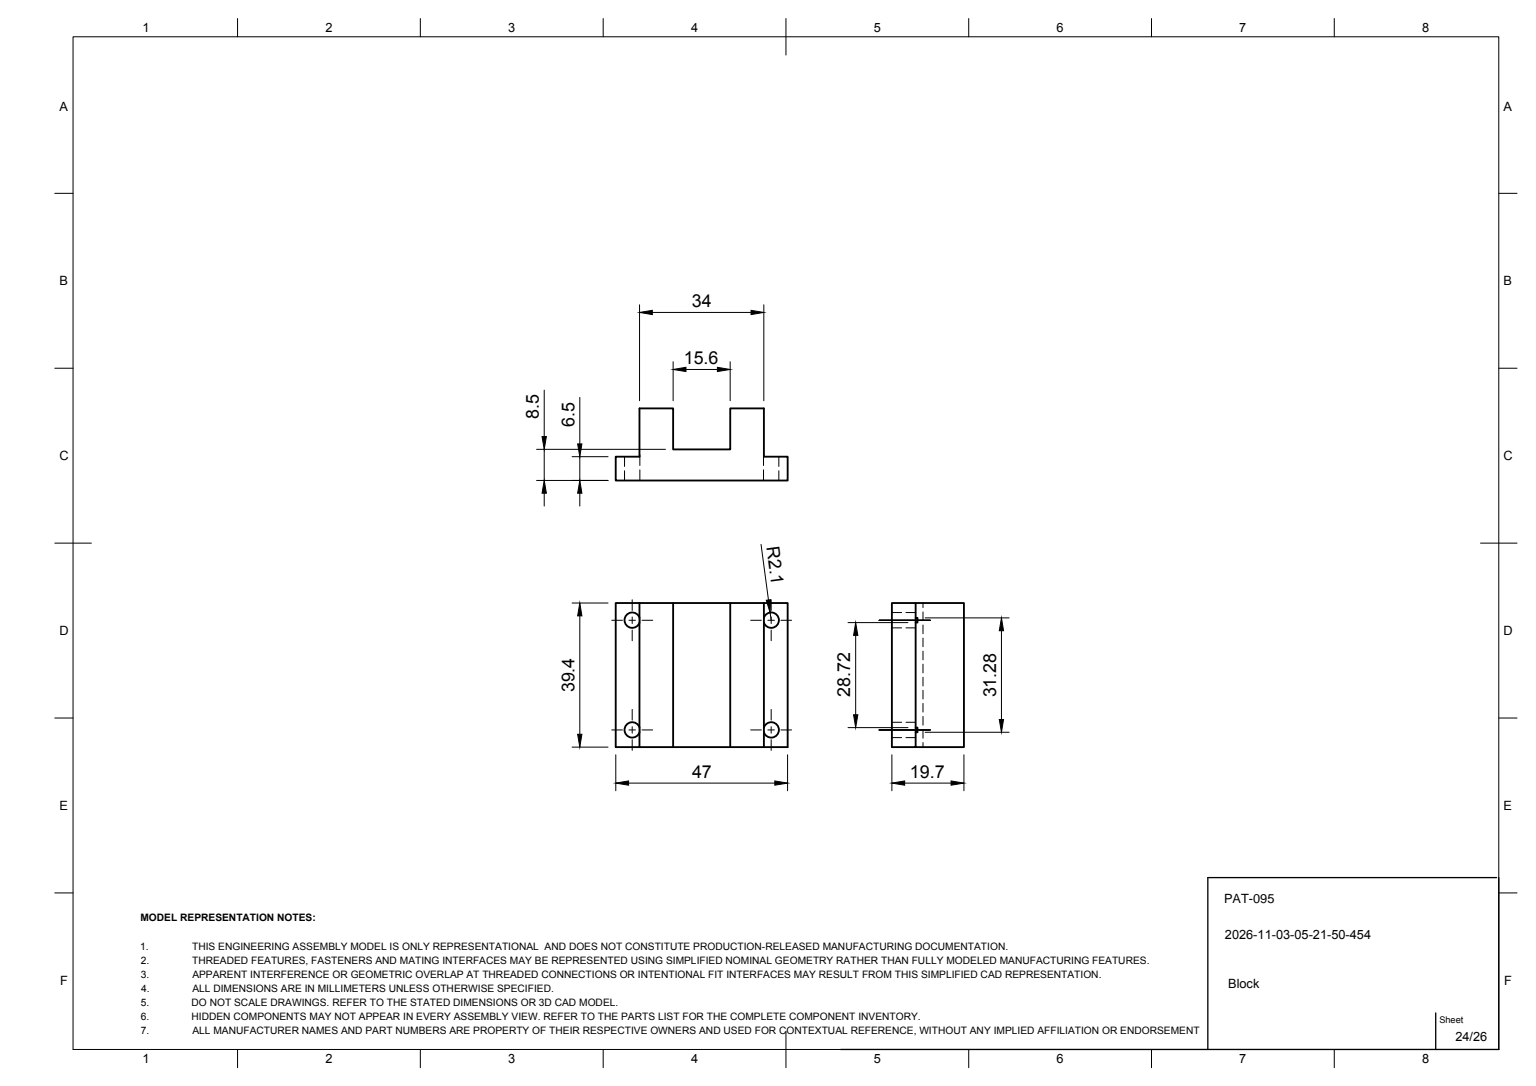
ISO-10303-21;
HEADER;
/* Generated by software containing ST-Developer
 * from STEP Tools, Inc. (www.steptools.com) 
 */

FILE_DESCRIPTION(
/* description */ ('Single-Axis Profile-Rail Linear Slide'),
/* implementation_level */ '2;1');

FILE_NAME(
/* name */ 'Block.step',
/* time_stamp */ '2026-10-27T10:47:43-07:00',
/* author */ (''),
/* organization */ (''),
/* preprocessor_version */ 'ST-DEVELOPER v20.2',
/* originating_system */ 'Autodesk Translation Framework v15.17.0.0',
/* authorisation */ '');

FILE_SCHEMA (('AUTOMOTIVE_DESIGN { 1 0 10303 214 3 1 1 }'));
ENDSEC;

DATA;
#10=MECHANICAL_DESIGN_GEOMETRIC_PRESENTATION_REPRESENTATION('',(#347),#14478);
#293=SHAPE_REPRESENTATION_RELATIONSHIP('SRR','None',#14625,#320);
#320=ADVANCED_BREP_SHAPE_REPRESENTATION('',(#372),#14469);
#347=STYLED_ITEM('',(#14810),#372);
#372=MANIFOLD_SOLID_BREP('Body1',#8609);
#455=FACE_BOUND('',#1734,.T.);
#456=FACE_BOUND('',#1735,.T.);
#457=FACE_BOUND('',#1736,.T.);
#458=FACE_BOUND('',#1737,.T.);
#763=PLANE('',#9394);
#764=PLANE('',#9400);
#765=PLANE('',#9406);
#766=PLANE('',#9412);
#767=PLANE('',#9418);
#768=PLANE('',#9419);
#769=PLANE('',#9420);
#770=PLANE('',#9421);
#771=PLANE('',#9422);
#772=PLANE('',#9423);
#773=PLANE('',#9424);
#774=PLANE('',#9425);
#775=PLANE('',#9426);
#776=PLANE('',#9427);
#777=PLANE('',#9428);
#778=PLANE('',#9429);
#779=PLANE('',#9430);
#780=PLANE('',#9431);
#1188=FACE_OUTER_BOUND('',#1720,.T.);
#1189=FACE_OUTER_BOUND('',#1721,.T.);
#1190=FACE_OUTER_BOUND('',#1722,.T.);
#1191=FACE_OUTER_BOUND('',#1723,.T.);
#1192=FACE_OUTER_BOUND('',#1724,.T.);
#1193=FACE_OUTER_BOUND('',#1725,.T.);
#1194=FACE_OUTER_BOUND('',#1726,.T.);
#1195=FACE_OUTER_BOUND('',#1727,.T.);
#1196=FACE_OUTER_BOUND('',#1728,.T.);
#1197=FACE_OUTER_BOUND('',#1729,.T.);
#1198=FACE_OUTER_BOUND('',#1730,.T.);
#1199=FACE_OUTER_BOUND('',#1731,.T.);
#1200=FACE_OUTER_BOUND('',#1732,.T.);
#1201=FACE_OUTER_BOUND('',#1733,.T.);
#1202=FACE_OUTER_BOUND('',#1738,.T.);
#1203=FACE_OUTER_BOUND('',#1739,.T.);
#1204=FACE_OUTER_BOUND('',#1740,.T.);
#1205=FACE_OUTER_BOUND('',#1741,.T.);
#1206=FACE_OUTER_BOUND('',#1742,.T.);
#1207=FACE_OUTER_BOUND('',#1743,.T.);
#1208=FACE_OUTER_BOUND('',#1744,.T.);
#1209=FACE_OUTER_BOUND('',#1745,.T.);
#1720=EDGE_LOOP('',(#7595,#7596));
#1721=EDGE_LOOP('',(#7597,#7598,#7599,#7600,#7601,#7602,#7603,#7604));
#1722=EDGE_LOOP('',(#7605,#7606));
#1723=EDGE_LOOP('',(#7607,#7608,#7609,#7610,#7611,#7612,#7613,#7614));
#1724=EDGE_LOOP('',(#7615,#7616));
#1725=EDGE_LOOP('',(#7617,#7618,#7619,#7620,#7621,#7622,#7623,#7624));
#1726=EDGE_LOOP('',(#7625,#7626));
#1727=EDGE_LOOP('',(#7627,#7628,#7629,#7630,#7631,#7632,#7633,#7634));
#1728=EDGE_LOOP('',(#7635,#7636,#7637,#7638,#7639,#7640,#7641,#7642,#7643,
#7644,#7645,#7646));
#1729=EDGE_LOOP('',(#7647,#7648,#7649,#7650,#7651,#7652,#7653,#7654,#7655,
#7656,#7657,#7658));
#1730=EDGE_LOOP('',(#7659,#7660,#7661,#7662,#7663,#7664,#7665,#7666,#7667,
#7668,#7669,#7670));
#1731=EDGE_LOOP('',(#7671,#7672,#7673,#7674,#7675,#7676,#7677,#7678,#7679,
#7680));
#1732=EDGE_LOOP('',(#7681,#7682,#7683,#7684));
#1733=EDGE_LOOP('',(#7685,#7686,#7687,#7688));
#1734=EDGE_LOOP('',(#7689));
#1735=EDGE_LOOP('',(#7690));
#1736=EDGE_LOOP('',(#7691));
#1737=EDGE_LOOP('',(#7692));
#1738=EDGE_LOOP('',(#7693,#7694,#7695,#7696));
#1739=EDGE_LOOP('',(#7697,#7698,#7699,#7700,#7701,#7702,#7703,#7704,#7705,
#7706));
#1740=EDGE_LOOP('',(#7707,#7708,#7709,#7710));
#1741=EDGE_LOOP('',(#7711,#7712,#7713,#7714));
#1742=EDGE_LOOP('',(#7715,#7716,#7717,#7718));
#1743=EDGE_LOOP('',(#7719,#7720,#7721,#7722));
#1744=EDGE_LOOP('',(#7723,#7724,#7725,#7726));
#1745=EDGE_LOOP('',(#7727,#7728,#7729,#7730,#7731,#7732,#7733,#7734,#7735,
#7736,#7737,#7738));
#2627=LINE('',#13853,#3598);
#2628=LINE('',#13857,#3599);
#2629=LINE('',#13861,#3600);
#2630=LINE('',#13865,#3601);
#2631=LINE('',#13869,#3602);
#2632=LINE('',#13873,#3603);
#2633=LINE('',#13877,#3604);
#2634=LINE('',#13881,#3605);
#2635=LINE('',#13885,#3606);
#2636=LINE('',#13889,#3607);
#2637=LINE('',#13893,#3608);
#2638=LINE('',#13897,#3609);
#2639=LINE('',#13901,#3610);
#2640=LINE('',#13905,#3611);
#2641=LINE('',#13909,#3612);
#2642=LINE('',#13913,#3613);
#2643=LINE('',#13915,#3614);
#2644=LINE('',#13917,#3615);
#2645=LINE('',#13919,#3616);
#2646=LINE('',#13921,#3617);
#2647=LINE('',#13923,#3618);
#2648=LINE('',#13924,#3619);
#2649=LINE('',#13926,#3620);
#2650=LINE('',#13928,#3621);
#2651=LINE('',#13930,#3622);
#2652=LINE('',#13932,#3623);
#2653=LINE('',#13934,#3624);
#2654=LINE('',#13935,#3625);
#2655=LINE('',#13938,#3626);
#2656=LINE('',#13940,#3627);
#2657=LINE('',#13942,#3628);
#2658=LINE('',#13944,#3629);
#2659=LINE('',#13945,#3630);
#2660=LINE('',#13947,#3631);
#2661=LINE('',#13949,#3632);
#2662=LINE('',#13951,#3633);
#2663=LINE('',#13953,#3634);
#2664=LINE('',#13954,#3635);
#2665=LINE('',#13957,#3636);
#2666=LINE('',#13958,#3637);
#2667=LINE('',#13961,#3638);
#2668=LINE('',#13962,#3639);
#2669=LINE('',#13965,#3640);
#2670=LINE('',#13966,#3641);
#2671=LINE('',#13969,#3642);
#2672=LINE('',#13970,#3643);
#2673=LINE('',#13972,#3644);
#2674=LINE('',#13975,#3645);
#2675=LINE('',#13976,#3646);
#2676=LINE('',#13979,#3647);
#2677=LINE('',#13980,#3648);
#2678=LINE('',#13983,#3649);
#2679=LINE('',#13984,#3650);
#2680=LINE('',#13987,#3651);
#2681=LINE('',#13988,#3652);
#2682=LINE('',#13990,#3653);
#3598=VECTOR('',#11360,1.);
#3599=VECTOR('',#11365,1.);
#3600=VECTOR('',#11368,0.21);
#3601=VECTOR('',#11373,1.);
#3602=VECTOR('',#11376,1.);
#3603=VECTOR('',#11381,1.);
#3604=VECTOR('',#11384,0.21);
#3605=VECTOR('',#11389,1.);
#3606=VECTOR('',#11392,1.);
#3607=VECTOR('',#11397,1.);
#3608=VECTOR('',#11400,0.21);
#3609=VECTOR('',#11405,1.);
#3610=VECTOR('',#11408,1.);
#3611=VECTOR('',#11413,1.);
#3612=VECTOR('',#11416,0.21);
#3613=VECTOR('',#11421,1.);
#3614=VECTOR('',#11424,1.);
#3615=VECTOR('',#11425,1.);
#3616=VECTOR('',#11426,1.);
#3617=VECTOR('',#11427,1.);
#3618=VECTOR('',#11428,1.);
#3619=VECTOR('',#11429,1.);
#3620=VECTOR('',#11432,1.);
#3621=VECTOR('',#11433,1.);
#3622=VECTOR('',#11434,1.);
#3623=VECTOR('',#11435,1.);
#3624=VECTOR('',#11436,1.);
#3625=VECTOR('',#11437,1.);
#3626=VECTOR('',#11440,1.);
#3627=VECTOR('',#11441,1.);
#3628=VECTOR('',#11442,1.);
#3629=VECTOR('',#11443,1.);
#3630=VECTOR('',#11444,1.);
#3631=VECTOR('',#11445,1.);
#3632=VECTOR('',#11446,1.);
#3633=VECTOR('',#11447,1.);
#3634=VECTOR('',#11448,1.);
#3635=VECTOR('',#11449,1.);
#3636=VECTOR('',#11452,1.);
#3637=VECTOR('',#11453,1.);
#3638=VECTOR('',#11456,1.);
#3639=VECTOR('',#11457,1.);
#3640=VECTOR('',#11460,1.);
#3641=VECTOR('',#11461,1.);
#3642=VECTOR('',#11464,1.);
#3643=VECTOR('',#11465,1.);
#3644=VECTOR('',#11468,1.);
#3645=VECTOR('',#11471,1.);
#3646=VECTOR('',#11472,1.);
#3647=VECTOR('',#11475,1.);
#3648=VECTOR('',#11476,1.);
#3649=VECTOR('',#11479,1.);
#3650=VECTOR('',#11480,1.);
#3651=VECTOR('',#11483,1.);
#3652=VECTOR('',#11484,1.);
#3653=VECTOR('',#11487,1.);
#3884=CIRCLE('',#9395,0.21);
#3885=CIRCLE('',#9397,0.21);
#3886=CIRCLE('',#9398,0.21);
#3887=CIRCLE('',#9399,0.21);
#3888=CIRCLE('',#9401,0.21);
#3889=CIRCLE('',#9403,0.21);
#3890=CIRCLE('',#9404,0.21);
#3891=CIRCLE('',#9405,0.21);
#3892=CIRCLE('',#9407,0.21);
#3893=CIRCLE('',#9409,0.21);
#3894=CIRCLE('',#9410,0.21);
#3895=CIRCLE('',#9411,0.21);
#3896=CIRCLE('',#9413,0.21);
#3897=CIRCLE('',#9415,0.21);
#3898=CIRCLE('',#9416,0.21);
#3899=CIRCLE('',#9417,0.21);
#4530=VERTEX_POINT('',#13851);
#4531=VERTEX_POINT('',#13852);
#4532=VERTEX_POINT('',#13856);
#4533=VERTEX_POINT('',#13858);
#4534=VERTEX_POINT('',#13860);
#4535=VERTEX_POINT('',#13863);
#4536=VERTEX_POINT('',#13867);
#4537=VERTEX_POINT('',#13868);
#4538=VERTEX_POINT('',#13872);
#4539=VERTEX_POINT('',#13874);
#4540=VERTEX_POINT('',#13876);
#4541=VERTEX_POINT('',#13879);
#4542=VERTEX_POINT('',#13883);
#4543=VERTEX_POINT('',#13884);
#4544=VERTEX_POINT('',#13888);
#4545=VERTEX_POINT('',#13890);
#4546=VERTEX_POINT('',#13892);
#4547=VERTEX_POINT('',#13895);
#4548=VERTEX_POINT('',#13899);
#4549=VERTEX_POINT('',#13900);
#4550=VERTEX_POINT('',#13904);
#4551=VERTEX_POINT('',#13906);
#4552=VERTEX_POINT('',#13908);
#4553=VERTEX_POINT('',#13911);
#4554=VERTEX_POINT('',#13916);
#4555=VERTEX_POINT('',#13918);
#4556=VERTEX_POINT('',#13920);
#4557=VERTEX_POINT('',#13922);
#4558=VERTEX_POINT('',#13927);
#4559=VERTEX_POINT('',#13929);
#4560=VERTEX_POINT('',#13931);
#4561=VERTEX_POINT('',#13933);
#4562=VERTEX_POINT('',#13937);
#4563=VERTEX_POINT('',#13939);
#4564=VERTEX_POINT('',#13941);
#4565=VERTEX_POINT('',#13943);
#4566=VERTEX_POINT('',#13946);
#4567=VERTEX_POINT('',#13948);
#4568=VERTEX_POINT('',#13950);
#4569=VERTEX_POINT('',#13952);
#4570=VERTEX_POINT('',#13956);
#4571=VERTEX_POINT('',#13960);
#4572=VERTEX_POINT('',#13964);
#4573=VERTEX_POINT('',#13968);
#4574=VERTEX_POINT('',#13974);
#4575=VERTEX_POINT('',#13978);
#4576=VERTEX_POINT('',#13982);
#4577=VERTEX_POINT('',#13986);
#5575=EDGE_CURVE('',#4530,#4531,#2627,.T.);
#5576=EDGE_CURVE('',#4530,#4531,#3884,.T.);
#5577=EDGE_CURVE('',#4532,#4530,#2628,.T.);
#5578=EDGE_CURVE('',#4533,#4532,#3885,.T.);
#5579=EDGE_CURVE('',#4533,#4534,#2629,.T.);
#5580=EDGE_CURVE('',#4534,#4534,#3886,.T.);
#5581=EDGE_CURVE('',#4535,#4533,#3887,.T.);
#5582=EDGE_CURVE('',#4531,#4535,#2630,.T.);
#5583=EDGE_CURVE('',#4536,#4537,#2631,.T.);
#5584=EDGE_CURVE('',#4536,#4537,#3888,.T.);
#5585=EDGE_CURVE('',#4538,#4536,#2632,.T.);
#5586=EDGE_CURVE('',#4539,#4538,#3889,.T.);
#5587=EDGE_CURVE('',#4539,#4540,#2633,.T.);
#5588=EDGE_CURVE('',#4540,#4540,#3890,.T.);
#5589=EDGE_CURVE('',#4541,#4539,#3891,.T.);
#5590=EDGE_CURVE('',#4537,#4541,#2634,.T.);
#5591=EDGE_CURVE('',#4542,#4543,#2635,.T.);
#5592=EDGE_CURVE('',#4542,#4543,#3892,.T.);
#5593=EDGE_CURVE('',#4544,#4542,#2636,.T.);
#5594=EDGE_CURVE('',#4545,#4544,#3893,.T.);
#5595=EDGE_CURVE('',#4545,#4546,#2637,.T.);
#5596=EDGE_CURVE('',#4546,#4546,#3894,.T.);
#5597=EDGE_CURVE('',#4547,#4545,#3895,.T.);
#5598=EDGE_CURVE('',#4543,#4547,#2638,.T.);
#5599=EDGE_CURVE('',#4548,#4549,#2639,.T.);
#5600=EDGE_CURVE('',#4548,#4549,#3896,.T.);
#5601=EDGE_CURVE('',#4550,#4548,#2640,.T.);
#5602=EDGE_CURVE('',#4551,#4550,#3897,.T.);
#5603=EDGE_CURVE('',#4551,#4552,#2641,.T.);
#5604=EDGE_CURVE('',#4552,#4552,#3898,.T.);
#5605=EDGE_CURVE('',#4553,#4551,#3899,.T.);
#5606=EDGE_CURVE('',#4549,#4553,#2642,.T.);
#5607=EDGE_CURVE('',#4535,#4544,#2643,.T.);
#5608=EDGE_CURVE('',#4547,#4554,#2644,.T.);
#5609=EDGE_CURVE('',#4555,#4554,#2645,.T.);
#5610=EDGE_CURVE('',#4555,#4556,#2646,.T.);
#5611=EDGE_CURVE('',#4557,#4556,#2647,.T.);
#5612=EDGE_CURVE('',#4557,#4532,#2648,.T.);
#5613=EDGE_CURVE('',#4541,#4550,#2649,.T.);
#5614=EDGE_CURVE('',#4553,#4558,#2650,.T.);
#5615=EDGE_CURVE('',#4559,#4558,#2651,.T.);
#5616=EDGE_CURVE('',#4560,#4559,#2652,.T.);
#5617=EDGE_CURVE('',#4561,#4560,#2653,.T.);
#5618=EDGE_CURVE('',#4561,#4538,#2654,.T.);
#5619=EDGE_CURVE('',#4554,#4562,#2655,.T.);
#5620=EDGE_CURVE('',#4562,#4563,#2656,.T.);
#5621=EDGE_CURVE('',#4563,#4564,#2657,.T.);
#5622=EDGE_CURVE('',#4564,#4565,#2658,.T.);
#5623=EDGE_CURVE('',#4565,#4561,#2659,.T.);
#5624=EDGE_CURVE('',#4560,#4566,#2660,.T.);
#5625=EDGE_CURVE('',#4566,#4567,#2661,.T.);
#5626=EDGE_CURVE('',#4567,#4568,#2662,.T.);
#5627=EDGE_CURVE('',#4568,#4569,#2663,.T.);
#5628=EDGE_CURVE('',#4569,#4555,#2664,.T.);
#5629=EDGE_CURVE('',#4570,#4557,#2665,.T.);
#5630=EDGE_CURVE('',#4562,#4570,#2666,.T.);
#5631=EDGE_CURVE('',#4571,#4570,#2667,.T.);
#5632=EDGE_CURVE('',#4563,#4571,#2668,.T.);
#5633=EDGE_CURVE('',#4572,#4571,#2669,.T.);
#5634=EDGE_CURVE('',#4564,#4572,#2670,.T.);
#5635=EDGE_CURVE('',#4573,#4572,#2671,.T.);
#5636=EDGE_CURVE('',#4565,#4573,#2672,.T.);
#5637=EDGE_CURVE('',#4558,#4573,#2673,.T.);
#5638=EDGE_CURVE('',#4574,#4559,#2674,.T.);
#5639=EDGE_CURVE('',#4566,#4574,#2675,.T.);
#5640=EDGE_CURVE('',#4575,#4574,#2676,.T.);
#5641=EDGE_CURVE('',#4567,#4575,#2677,.T.);
#5642=EDGE_CURVE('',#4576,#4575,#2678,.T.);
#5643=EDGE_CURVE('',#4568,#4576,#2679,.T.);
#5644=EDGE_CURVE('',#4577,#4576,#2680,.T.);
#5645=EDGE_CURVE('',#4569,#4577,#2681,.T.);
#5646=EDGE_CURVE('',#4556,#4577,#2682,.T.);
#7595=ORIENTED_EDGE('',*,*,#5575,.F.);
#7596=ORIENTED_EDGE('',*,*,#5576,.T.);
#7597=ORIENTED_EDGE('',*,*,#5577,.F.);
#7598=ORIENTED_EDGE('',*,*,#5578,.F.);
#7599=ORIENTED_EDGE('',*,*,#5579,.T.);
#7600=ORIENTED_EDGE('',*,*,#5580,.F.);
#7601=ORIENTED_EDGE('',*,*,#5579,.F.);
#7602=ORIENTED_EDGE('',*,*,#5581,.F.);
#7603=ORIENTED_EDGE('',*,*,#5582,.F.);
#7604=ORIENTED_EDGE('',*,*,#5576,.F.);
#7605=ORIENTED_EDGE('',*,*,#5583,.F.);
#7606=ORIENTED_EDGE('',*,*,#5584,.T.);
#7607=ORIENTED_EDGE('',*,*,#5585,.F.);
#7608=ORIENTED_EDGE('',*,*,#5586,.F.);
#7609=ORIENTED_EDGE('',*,*,#5587,.T.);
#7610=ORIENTED_EDGE('',*,*,#5588,.F.);
#7611=ORIENTED_EDGE('',*,*,#5587,.F.);
#7612=ORIENTED_EDGE('',*,*,#5589,.F.);
#7613=ORIENTED_EDGE('',*,*,#5590,.F.);
#7614=ORIENTED_EDGE('',*,*,#5584,.F.);
#7615=ORIENTED_EDGE('',*,*,#5591,.F.);
#7616=ORIENTED_EDGE('',*,*,#5592,.T.);
#7617=ORIENTED_EDGE('',*,*,#5593,.F.);
#7618=ORIENTED_EDGE('',*,*,#5594,.F.);
#7619=ORIENTED_EDGE('',*,*,#5595,.T.);
#7620=ORIENTED_EDGE('',*,*,#5596,.F.);
#7621=ORIENTED_EDGE('',*,*,#5595,.F.);
#7622=ORIENTED_EDGE('',*,*,#5597,.F.);
#7623=ORIENTED_EDGE('',*,*,#5598,.F.);
#7624=ORIENTED_EDGE('',*,*,#5592,.F.);
#7625=ORIENTED_EDGE('',*,*,#5599,.F.);
#7626=ORIENTED_EDGE('',*,*,#5600,.T.);
#7627=ORIENTED_EDGE('',*,*,#5601,.F.);
#7628=ORIENTED_EDGE('',*,*,#5602,.F.);
#7629=ORIENTED_EDGE('',*,*,#5603,.T.);
#7630=ORIENTED_EDGE('',*,*,#5604,.F.);
#7631=ORIENTED_EDGE('',*,*,#5603,.F.);
#7632=ORIENTED_EDGE('',*,*,#5605,.F.);
#7633=ORIENTED_EDGE('',*,*,#5606,.F.);
#7634=ORIENTED_EDGE('',*,*,#5600,.F.);
#7635=ORIENTED_EDGE('',*,*,#5577,.T.);
#7636=ORIENTED_EDGE('',*,*,#5575,.T.);
#7637=ORIENTED_EDGE('',*,*,#5582,.T.);
#7638=ORIENTED_EDGE('',*,*,#5607,.T.);
#7639=ORIENTED_EDGE('',*,*,#5593,.T.);
#7640=ORIENTED_EDGE('',*,*,#5591,.T.);
#7641=ORIENTED_EDGE('',*,*,#5598,.T.);
#7642=ORIENTED_EDGE('',*,*,#5608,.T.);
#7643=ORIENTED_EDGE('',*,*,#5609,.F.);
#7644=ORIENTED_EDGE('',*,*,#5610,.T.);
#7645=ORIENTED_EDGE('',*,*,#5611,.F.);
#7646=ORIENTED_EDGE('',*,*,#5612,.T.);
#7647=ORIENTED_EDGE('',*,*,#5585,.T.);
#7648=ORIENTED_EDGE('',*,*,#5583,.T.);
#7649=ORIENTED_EDGE('',*,*,#5590,.T.);
#7650=ORIENTED_EDGE('',*,*,#5613,.T.);
#7651=ORIENTED_EDGE('',*,*,#5601,.T.);
#7652=ORIENTED_EDGE('',*,*,#5599,.T.);
#7653=ORIENTED_EDGE('',*,*,#5606,.T.);
#7654=ORIENTED_EDGE('',*,*,#5614,.T.);
#7655=ORIENTED_EDGE('',*,*,#5615,.F.);
#7656=ORIENTED_EDGE('',*,*,#5616,.F.);
#7657=ORIENTED_EDGE('',*,*,#5617,.F.);
#7658=ORIENTED_EDGE('',*,*,#5618,.T.);
#7659=ORIENTED_EDGE('',*,*,#5609,.T.);
#7660=ORIENTED_EDGE('',*,*,#5619,.T.);
#7661=ORIENTED_EDGE('',*,*,#5620,.T.);
#7662=ORIENTED_EDGE('',*,*,#5621,.T.);
#7663=ORIENTED_EDGE('',*,*,#5622,.T.);
#7664=ORIENTED_EDGE('',*,*,#5623,.T.);
#7665=ORIENTED_EDGE('',*,*,#5617,.T.);
#7666=ORIENTED_EDGE('',*,*,#5624,.T.);
#7667=ORIENTED_EDGE('',*,*,#5625,.T.);
#7668=ORIENTED_EDGE('',*,*,#5626,.T.);
#7669=ORIENTED_EDGE('',*,*,#5627,.T.);
#7670=ORIENTED_EDGE('',*,*,#5628,.T.);
#7671=ORIENTED_EDGE('',*,*,#5581,.T.);
#7672=ORIENTED_EDGE('',*,*,#5578,.T.);
#7673=ORIENTED_EDGE('',*,*,#5612,.F.);
#7674=ORIENTED_EDGE('',*,*,#5629,.F.);
#7675=ORIENTED_EDGE('',*,*,#5630,.F.);
#7676=ORIENTED_EDGE('',*,*,#5619,.F.);
#7677=ORIENTED_EDGE('',*,*,#5608,.F.);
#7678=ORIENTED_EDGE('',*,*,#5597,.T.);
#7679=ORIENTED_EDGE('',*,*,#5594,.T.);
#7680=ORIENTED_EDGE('',*,*,#5607,.F.);
#7681=ORIENTED_EDGE('',*,*,#5630,.T.);
#7682=ORIENTED_EDGE('',*,*,#5631,.F.);
#7683=ORIENTED_EDGE('',*,*,#5632,.F.);
#7684=ORIENTED_EDGE('',*,*,#5620,.F.);
#7685=ORIENTED_EDGE('',*,*,#5632,.T.);
#7686=ORIENTED_EDGE('',*,*,#5633,.F.);
#7687=ORIENTED_EDGE('',*,*,#5634,.F.);
#7688=ORIENTED_EDGE('',*,*,#5621,.F.);
#7689=ORIENTED_EDGE('',*,*,#5580,.T.);
#7690=ORIENTED_EDGE('',*,*,#5588,.T.);
#7691=ORIENTED_EDGE('',*,*,#5596,.T.);
#7692=ORIENTED_EDGE('',*,*,#5604,.T.);
#7693=ORIENTED_EDGE('',*,*,#5634,.T.);
#7694=ORIENTED_EDGE('',*,*,#5635,.F.);
#7695=ORIENTED_EDGE('',*,*,#5636,.F.);
#7696=ORIENTED_EDGE('',*,*,#5622,.F.);
#7697=ORIENTED_EDGE('',*,*,#5589,.T.);
#7698=ORIENTED_EDGE('',*,*,#5586,.T.);
#7699=ORIENTED_EDGE('',*,*,#5618,.F.);
#7700=ORIENTED_EDGE('',*,*,#5623,.F.);
#7701=ORIENTED_EDGE('',*,*,#5636,.T.);
#7702=ORIENTED_EDGE('',*,*,#5637,.F.);
#7703=ORIENTED_EDGE('',*,*,#5614,.F.);
#7704=ORIENTED_EDGE('',*,*,#5605,.T.);
#7705=ORIENTED_EDGE('',*,*,#5602,.T.);
#7706=ORIENTED_EDGE('',*,*,#5613,.F.);
#7707=ORIENTED_EDGE('',*,*,#5616,.T.);
#7708=ORIENTED_EDGE('',*,*,#5638,.F.);
#7709=ORIENTED_EDGE('',*,*,#5639,.F.);
#7710=ORIENTED_EDGE('',*,*,#5624,.F.);
#7711=ORIENTED_EDGE('',*,*,#5639,.T.);
#7712=ORIENTED_EDGE('',*,*,#5640,.F.);
#7713=ORIENTED_EDGE('',*,*,#5641,.F.);
#7714=ORIENTED_EDGE('',*,*,#5625,.F.);
#7715=ORIENTED_EDGE('',*,*,#5641,.T.);
#7716=ORIENTED_EDGE('',*,*,#5642,.F.);
#7717=ORIENTED_EDGE('',*,*,#5643,.F.);
#7718=ORIENTED_EDGE('',*,*,#5626,.F.);
#7719=ORIENTED_EDGE('',*,*,#5643,.T.);
#7720=ORIENTED_EDGE('',*,*,#5644,.F.);
#7721=ORIENTED_EDGE('',*,*,#5645,.F.);
#7722=ORIENTED_EDGE('',*,*,#5627,.F.);
#7723=ORIENTED_EDGE('',*,*,#5645,.T.);
#7724=ORIENTED_EDGE('',*,*,#5646,.F.);
#7725=ORIENTED_EDGE('',*,*,#5610,.F.);
#7726=ORIENTED_EDGE('',*,*,#5628,.F.);
#7727=ORIENTED_EDGE('',*,*,#5611,.T.);
#7728=ORIENTED_EDGE('',*,*,#5646,.T.);
#7729=ORIENTED_EDGE('',*,*,#5644,.T.);
#7730=ORIENTED_EDGE('',*,*,#5642,.T.);
#7731=ORIENTED_EDGE('',*,*,#5640,.T.);
#7732=ORIENTED_EDGE('',*,*,#5638,.T.);
#7733=ORIENTED_EDGE('',*,*,#5615,.T.);
#7734=ORIENTED_EDGE('',*,*,#5637,.T.);
#7735=ORIENTED_EDGE('',*,*,#5635,.T.);
#7736=ORIENTED_EDGE('',*,*,#5633,.T.);
#7737=ORIENTED_EDGE('',*,*,#5631,.T.);
#7738=ORIENTED_EDGE('',*,*,#5629,.T.);
#8118=CYLINDRICAL_SURFACE('',#9396,0.21);
#8119=CYLINDRICAL_SURFACE('',#9402,0.21);
#8120=CYLINDRICAL_SURFACE('',#9408,0.21);
#8121=CYLINDRICAL_SURFACE('',#9414,0.21);
#8482=ADVANCED_FACE('',(#1188),#763,.T.);
#8483=ADVANCED_FACE('',(#1189),#8118,.F.);
#8484=ADVANCED_FACE('',(#1190),#764,.T.);
#8485=ADVANCED_FACE('',(#1191),#8119,.F.);
#8486=ADVANCED_FACE('',(#1192),#765,.T.);
#8487=ADVANCED_FACE('',(#1193),#8120,.F.);
#8488=ADVANCED_FACE('',(#1194),#766,.T.);
#8489=ADVANCED_FACE('',(#1195),#8121,.F.);
#8490=ADVANCED_FACE('',(#1196),#767,.T.);
#8491=ADVANCED_FACE('',(#1197),#768,.T.);
#8492=ADVANCED_FACE('',(#1198),#769,.T.);
#8493=ADVANCED_FACE('',(#1199),#770,.T.);
#8494=ADVANCED_FACE('',(#1200),#771,.T.);
#8495=ADVANCED_FACE('',(#1201,#455,#456,#457,#458),#772,.T.);
#8496=ADVANCED_FACE('',(#1202),#773,.T.);
#8497=ADVANCED_FACE('',(#1203),#774,.T.);
#8498=ADVANCED_FACE('',(#1204),#775,.T.);
#8499=ADVANCED_FACE('',(#1205),#776,.T.);
#8500=ADVANCED_FACE('',(#1206),#777,.T.);
#8501=ADVANCED_FACE('',(#1207),#778,.T.);
#8502=ADVANCED_FACE('',(#1208),#779,.T.);
#8503=ADVANCED_FACE('',(#1209),#780,.T.);
#8609=CLOSED_SHELL('',(#8482,#8483,#8484,#8485,#8486,#8487,#8488,#8489,
#8490,#8491,#8492,#8493,#8494,#8495,#8496,#8497,#8498,#8499,#8500,#8501,
#8502,#8503));
#9393=AXIS2_PLACEMENT_3D('',#13849,#11356,#11357);
#9394=AXIS2_PLACEMENT_3D('',#13850,#11358,#11359);
#9395=AXIS2_PLACEMENT_3D('',#13854,#11361,#11362);
#9396=AXIS2_PLACEMENT_3D('',#13855,#11363,#11364);
#9397=AXIS2_PLACEMENT_3D('',#13859,#11366,#11367);
#9398=AXIS2_PLACEMENT_3D('',#13862,#11369,#11370);
#9399=AXIS2_PLACEMENT_3D('',#13864,#11371,#11372);
#9400=AXIS2_PLACEMENT_3D('',#13866,#11374,#11375);
#9401=AXIS2_PLACEMENT_3D('',#13870,#11377,#11378);
#9402=AXIS2_PLACEMENT_3D('',#13871,#11379,#11380);
#9403=AXIS2_PLACEMENT_3D('',#13875,#11382,#11383);
#9404=AXIS2_PLACEMENT_3D('',#13878,#11385,#11386);
#9405=AXIS2_PLACEMENT_3D('',#13880,#11387,#11388);
#9406=AXIS2_PLACEMENT_3D('',#13882,#11390,#11391);
#9407=AXIS2_PLACEMENT_3D('',#13886,#11393,#11394);
#9408=AXIS2_PLACEMENT_3D('',#13887,#11395,#11396);
#9409=AXIS2_PLACEMENT_3D('',#13891,#11398,#11399);
#9410=AXIS2_PLACEMENT_3D('',#13894,#11401,#11402);
#9411=AXIS2_PLACEMENT_3D('',#13896,#11403,#11404);
#9412=AXIS2_PLACEMENT_3D('',#13898,#11406,#11407);
#9413=AXIS2_PLACEMENT_3D('',#13902,#11409,#11410);
#9414=AXIS2_PLACEMENT_3D('',#13903,#11411,#11412);
#9415=AXIS2_PLACEMENT_3D('',#13907,#11414,#11415);
#9416=AXIS2_PLACEMENT_3D('',#13910,#11417,#11418);
#9417=AXIS2_PLACEMENT_3D('',#13912,#11419,#11420);
#9418=AXIS2_PLACEMENT_3D('',#13914,#11422,#11423);
#9419=AXIS2_PLACEMENT_3D('',#13925,#11430,#11431);
#9420=AXIS2_PLACEMENT_3D('',#13936,#11438,#11439);
#9421=AXIS2_PLACEMENT_3D('',#13955,#11450,#11451);
#9422=AXIS2_PLACEMENT_3D('',#13959,#11454,#11455);
#9423=AXIS2_PLACEMENT_3D('',#13963,#11458,#11459);
#9424=AXIS2_PLACEMENT_3D('',#13967,#11462,#11463);
#9425=AXIS2_PLACEMENT_3D('',#13971,#11466,#11467);
#9426=AXIS2_PLACEMENT_3D('',#13973,#11469,#11470);
#9427=AXIS2_PLACEMENT_3D('',#13977,#11473,#11474);
#9428=AXIS2_PLACEMENT_3D('',#13981,#11477,#11478);
#9429=AXIS2_PLACEMENT_3D('',#13985,#11481,#11482);
#9430=AXIS2_PLACEMENT_3D('',#13989,#11485,#11486);
#9431=AXIS2_PLACEMENT_3D('',#13991,#11488,#11489);
#11356=DIRECTION('axis',(0.,0.,1.));
#11357=DIRECTION('refdir',(1.,0.,0.));
#11358=DIRECTION('center_axis',(0.,0.,1.));
#11359=DIRECTION('ref_axis',(1.,0.,0.));
#11360=DIRECTION('',(-1.,0.,0.));
#11361=DIRECTION('center_axis',(0.,0.,1.));
#11362=DIRECTION('ref_axis',(1.,0.,0.));
#11363=DIRECTION('center_axis',(0.,0.,1.));
#11364=DIRECTION('ref_axis',(1.,0.,0.));
#11365=DIRECTION('',(0.,0.,-1.));
#11366=DIRECTION('center_axis',(0.,0.,1.));
#11367=DIRECTION('ref_axis',(1.,0.,0.));
#11368=DIRECTION('',(0.,0.,1.));
#11369=DIRECTION('center_axis',(0.,0.,-1.));
#11370=DIRECTION('ref_axis',(1.,0.,0.));
#11371=DIRECTION('center_axis',(0.,0.,1.));
#11372=DIRECTION('ref_axis',(1.,0.,0.));
#11373=DIRECTION('',(0.,0.,1.));
#11374=DIRECTION('center_axis',(0.,0.,1.));
#11375=DIRECTION('ref_axis',(1.,0.,0.));
#11376=DIRECTION('',(1.,0.,0.));
#11377=DIRECTION('center_axis',(0.,0.,1.));
#11378=DIRECTION('ref_axis',(1.,0.,0.));
#11379=DIRECTION('center_axis',(0.,0.,1.));
#11380=DIRECTION('ref_axis',(1.,0.,0.));
#11381=DIRECTION('',(0.,0.,-1.));
#11382=DIRECTION('center_axis',(0.,0.,1.));
#11383=DIRECTION('ref_axis',(1.,0.,0.));
#11384=DIRECTION('',(0.,0.,1.));
#11385=DIRECTION('center_axis',(0.,0.,-1.));
#11386=DIRECTION('ref_axis',(1.,0.,0.));
#11387=DIRECTION('center_axis',(0.,0.,1.));
#11388=DIRECTION('ref_axis',(1.,0.,0.));
#11389=DIRECTION('',(0.,0.,1.));
#11390=DIRECTION('center_axis',(0.,0.,1.));
#11391=DIRECTION('ref_axis',(1.,0.,0.));
#11392=DIRECTION('',(-1.,0.,0.));
#11393=DIRECTION('center_axis',(0.,0.,1.));
#11394=DIRECTION('ref_axis',(1.,0.,0.));
#11395=DIRECTION('center_axis',(0.,0.,1.));
#11396=DIRECTION('ref_axis',(1.,0.,0.));
#11397=DIRECTION('',(0.,0.,-1.));
#11398=DIRECTION('center_axis',(0.,0.,1.));
#11399=DIRECTION('ref_axis',(1.,0.,0.));
#11400=DIRECTION('',(0.,0.,1.));
#11401=DIRECTION('center_axis',(0.,0.,-1.));
#11402=DIRECTION('ref_axis',(1.,0.,0.));
#11403=DIRECTION('center_axis',(0.,0.,1.));
#11404=DIRECTION('ref_axis',(1.,0.,0.));
#11405=DIRECTION('',(0.,0.,1.));
#11406=DIRECTION('center_axis',(0.,0.,1.));
#11407=DIRECTION('ref_axis',(1.,0.,0.));
#11408=DIRECTION('',(1.,0.,0.));
#11409=DIRECTION('center_axis',(0.,0.,1.));
#11410=DIRECTION('ref_axis',(1.,0.,0.));
#11411=DIRECTION('center_axis',(0.,0.,1.));
#11412=DIRECTION('ref_axis',(1.,0.,0.));
#11413=DIRECTION('',(0.,0.,-1.));
#11414=DIRECTION('center_axis',(0.,0.,1.));
#11415=DIRECTION('ref_axis',(1.,0.,0.));
#11416=DIRECTION('',(0.,0.,1.));
#11417=DIRECTION('center_axis',(0.,0.,-1.));
#11418=DIRECTION('ref_axis',(1.,0.,0.));
#11419=DIRECTION('center_axis',(0.,0.,1.));
#11420=DIRECTION('ref_axis',(1.,0.,0.));
#11421=DIRECTION('',(0.,0.,1.));
#11422=DIRECTION('center_axis',(0.,-1.,0.));
#11423=DIRECTION('ref_axis',(0.,0.,-1.));
#11424=DIRECTION('',(-1.,0.,0.));
#11425=DIRECTION('',(-1.,0.,0.));
#11426=DIRECTION('',(0.,0.,1.));
#11427=DIRECTION('',(1.,0.,0.));
#11428=DIRECTION('',(0.,0.,-1.));
#11429=DIRECTION('',(-1.,0.,0.));
#11430=DIRECTION('center_axis',(0.,1.,0.));
#11431=DIRECTION('ref_axis',(0.,0.,1.));
#11432=DIRECTION('',(1.,0.,0.));
#11433=DIRECTION('',(1.,0.,0.));
#11434=DIRECTION('',(0.,0.,1.));
#11435=DIRECTION('',(1.,0.,0.));
#11436=DIRECTION('',(0.,0.,-1.));
#11437=DIRECTION('',(1.,0.,0.));
#11438=DIRECTION('center_axis',(-1.,0.,0.));
#11439=DIRECTION('ref_axis',(0.,0.,1.));
#11440=DIRECTION('',(0.,-1.,0.));
#11441=DIRECTION('',(0.,0.,1.));
#11442=DIRECTION('',(0.,1.,0.));
#11443=DIRECTION('',(0.,0.,-1.));
#11444=DIRECTION('',(0.,-1.,0.));
#11445=DIRECTION('',(0.,-1.,0.));
#11446=DIRECTION('',(0.,0.,1.));
#11447=DIRECTION('',(0.,-1.,0.));
#11448=DIRECTION('',(0.,0.,-1.));
#11449=DIRECTION('',(0.,-1.,0.));
#11450=DIRECTION('center_axis',(0.,0.,-1.));
#11451=DIRECTION('ref_axis',(0.,1.,0.));
#11452=DIRECTION('',(0.,1.,0.));
#11453=DIRECTION('',(1.,0.,0.));
#11454=DIRECTION('center_axis',(0.,-1.,0.));
#11455=DIRECTION('ref_axis',(0.,0.,-1.));
#11456=DIRECTION('',(0.,0.,-1.));
#11457=DIRECTION('',(1.,0.,0.));
#11458=DIRECTION('center_axis',(0.,0.,1.));
#11459=DIRECTION('ref_axis',(0.,-1.,0.));
#11460=DIRECTION('',(0.,-1.,0.));
#11461=DIRECTION('',(1.,0.,0.));
#11462=DIRECTION('center_axis',(0.,1.,0.));
#11463=DIRECTION('ref_axis',(0.,0.,1.));
#11464=DIRECTION('',(0.,0.,1.));
#11465=DIRECTION('',(1.,0.,0.));
#11466=DIRECTION('center_axis',(0.,0.,-1.));
#11467=DIRECTION('ref_axis',(0.,1.,0.));
#11468=DIRECTION('',(0.,1.,0.));
#11469=DIRECTION('center_axis',(0.,0.,-1.));
#11470=DIRECTION('ref_axis',(0.,1.,0.));
#11471=DIRECTION('',(0.,1.,0.));
#11472=DIRECTION('',(1.,0.,0.));
#11473=DIRECTION('center_axis',(0.,-1.,0.));
#11474=DIRECTION('ref_axis',(0.,0.,-1.));
#11475=DIRECTION('',(0.,0.,-1.));
#11476=DIRECTION('',(1.,0.,0.));
#11477=DIRECTION('center_axis',(0.,0.,-1.));
#11478=DIRECTION('ref_axis',(0.,1.,0.));
#11479=DIRECTION('',(0.,1.,0.));
#11480=DIRECTION('',(1.,0.,0.));
#11481=DIRECTION('center_axis',(0.,1.,0.));
#11482=DIRECTION('ref_axis',(0.,0.,1.));
#11483=DIRECTION('',(0.,0.,1.));
#11484=DIRECTION('',(1.,0.,0.));
#11485=DIRECTION('center_axis',(0.,0.,-1.));
#11486=DIRECTION('ref_axis',(0.,1.,0.));
#11487=DIRECTION('',(0.,1.,0.));
#11488=DIRECTION('center_axis',(1.,0.,0.));
#11489=DIRECTION('ref_axis',(0.,0.,-1.));
#13849=CARTESIAN_POINT('',(0.,0.,0.));
#13850=CARTESIAN_POINT('Origin',(1.5,-1.9,1.7));
#13851=CARTESIAN_POINT('',(1.56403124237433,-1.7,1.7));
#13852=CARTESIAN_POINT('',(1.43596875762567,-1.7,1.7));
#13853=CARTESIAN_POINT('',(0.75,-1.7,1.7));
#13854=CARTESIAN_POINT('Origin',(1.5,-1.9,1.7));
#13855=CARTESIAN_POINT('Origin',(1.5,-1.9,1.7));
#13856=CARTESIAN_POINT('',(1.56403124237433,-1.7,1.75));
#13857=CARTESIAN_POINT('',(1.56403124237433,-1.7,1.7));
#13858=CARTESIAN_POINT('',(1.29,-1.9,1.75));
#13859=CARTESIAN_POINT('Origin',(1.5,-1.9,1.75));
#13860=CARTESIAN_POINT('',(1.29,-1.9,2.4));
#13861=CARTESIAN_POINT('',(1.29,-1.9,1.7));
#13862=CARTESIAN_POINT('Origin',(1.5,-1.9,2.4));
#13863=CARTESIAN_POINT('',(1.43596875762567,-1.7,1.75));
#13864=CARTESIAN_POINT('Origin',(1.5,-1.9,1.75));
#13865=CARTESIAN_POINT('',(1.43596875762567,-1.7,1.7));
#13866=CARTESIAN_POINT('Origin',(-1.5,1.9,1.7));
#13867=CARTESIAN_POINT('',(-1.56403124237433,1.7,1.7));
#13868=CARTESIAN_POINT('',(-1.43596875762567,1.7,1.7));
#13869=CARTESIAN_POINT('',(-0.75,1.7,1.7));
#13870=CARTESIAN_POINT('Origin',(-1.5,1.9,1.7));
#13871=CARTESIAN_POINT('Origin',(-1.5,1.9,1.7));
#13872=CARTESIAN_POINT('',(-1.56403124237433,1.7,1.75));
#13873=CARTESIAN_POINT('',(-1.56403124237433,1.7,1.7));
#13874=CARTESIAN_POINT('',(-1.71,1.9,1.75));
#13875=CARTESIAN_POINT('Origin',(-1.5,1.9,1.75));
#13876=CARTESIAN_POINT('',(-1.71,1.9,2.4));
#13877=CARTESIAN_POINT('',(-1.71,1.9,1.7));
#13878=CARTESIAN_POINT('Origin',(-1.5,1.9,2.4));
#13879=CARTESIAN_POINT('',(-1.43596875762567,1.7,1.75));
#13880=CARTESIAN_POINT('Origin',(-1.5,1.9,1.75));
#13881=CARTESIAN_POINT('',(-1.43596875762567,1.7,1.7));
#13882=CARTESIAN_POINT('Origin',(-1.5,-1.9,1.7));
#13883=CARTESIAN_POINT('',(-1.43596875762567,-1.7,1.7));
#13884=CARTESIAN_POINT('',(-1.56403124237433,-1.7,1.7));
#13885=CARTESIAN_POINT('',(-0.75,-1.7,1.7));
#13886=CARTESIAN_POINT('Origin',(-1.5,-1.9,1.7));
#13887=CARTESIAN_POINT('Origin',(-1.5,-1.9,1.7));
#13888=CARTESIAN_POINT('',(-1.43596875762567,-1.7,1.75));
#13889=CARTESIAN_POINT('',(-1.43596875762567,-1.7,1.7));
#13890=CARTESIAN_POINT('',(-1.71,-1.9,1.75));
#13891=CARTESIAN_POINT('Origin',(-1.5,-1.9,1.75));
#13892=CARTESIAN_POINT('',(-1.71,-1.9,2.4));
#13893=CARTESIAN_POINT('',(-1.71,-1.9,1.7));
#13894=CARTESIAN_POINT('Origin',(-1.5,-1.9,2.4));
#13895=CARTESIAN_POINT('',(-1.56403124237433,-1.7,1.75));
#13896=CARTESIAN_POINT('Origin',(-1.5,-1.9,1.75));
#13897=CARTESIAN_POINT('',(-1.56403124237433,-1.7,1.7));
#13898=CARTESIAN_POINT('Origin',(1.5,1.9,1.7));
#13899=CARTESIAN_POINT('',(1.43596875762567,1.7,1.7));
#13900=CARTESIAN_POINT('',(1.56403124237433,1.7,1.7));
#13901=CARTESIAN_POINT('',(0.75,1.7,1.7));
#13902=CARTESIAN_POINT('Origin',(1.5,1.9,1.7));
#13903=CARTESIAN_POINT('Origin',(1.5,1.9,1.7));
#13904=CARTESIAN_POINT('',(1.43596875762567,1.7,1.75));
#13905=CARTESIAN_POINT('',(1.43596875762567,1.7,1.7));
#13906=CARTESIAN_POINT('',(1.29,1.9,1.75));
#13907=CARTESIAN_POINT('Origin',(1.5,1.9,1.75));
#13908=CARTESIAN_POINT('',(1.29,1.9,2.4));
#13909=CARTESIAN_POINT('',(1.29,1.9,1.7));
#13910=CARTESIAN_POINT('Origin',(1.5,1.9,2.4));
#13911=CARTESIAN_POINT('',(1.56403124237433,1.7,1.75));
#13912=CARTESIAN_POINT('Origin',(1.5,1.9,1.75));
#13913=CARTESIAN_POINT('',(1.56403124237433,1.7,1.7));
#13914=CARTESIAN_POINT('Origin',(0.,-1.7,1.75));
#13915=CARTESIAN_POINT('',(0.,-1.7,1.75));
#13916=CARTESIAN_POINT('',(-1.97,-1.7,1.75));
#13917=CARTESIAN_POINT('',(0.,-1.7,1.75));
#13918=CARTESIAN_POINT('',(-1.97,-1.7,0.43));
#13919=CARTESIAN_POINT('',(-1.97,-1.7,1.75));
#13920=CARTESIAN_POINT('',(1.97,-1.7,0.43));
#13921=CARTESIAN_POINT('',(0.,-1.7,0.43));
#13922=CARTESIAN_POINT('',(1.97,-1.7,1.75));
#13923=CARTESIAN_POINT('',(1.97,-1.7,1.75));
#13924=CARTESIAN_POINT('',(0.,-1.7,1.75));
#13925=CARTESIAN_POINT('Origin',(0.,1.7,0.43));
#13926=CARTESIAN_POINT('',(0.,1.7,1.75));
#13927=CARTESIAN_POINT('',(1.97,1.7,1.75));
#13928=CARTESIAN_POINT('',(0.,1.7,1.75));
#13929=CARTESIAN_POINT('',(1.97,1.7,0.43));
#13930=CARTESIAN_POINT('',(1.97,1.7,0.43));
#13931=CARTESIAN_POINT('',(-1.97,1.7,0.43));
#13932=CARTESIAN_POINT('',(0.,1.7,0.43));
#13933=CARTESIAN_POINT('',(-1.97,1.7,1.75));
#13934=CARTESIAN_POINT('',(-1.97,1.7,0.43));
#13935=CARTESIAN_POINT('',(0.,1.7,1.75));
#13936=CARTESIAN_POINT('Origin',(-1.97,0.,1.415));
#13937=CARTESIAN_POINT('',(-1.97,-2.35,1.75));
#13938=CARTESIAN_POINT('',(-1.97,-2.35,1.75));
#13939=CARTESIAN_POINT('',(-1.97,-2.35,2.4));
#13940=CARTESIAN_POINT('',(-1.97,-2.35,2.4));
#13941=CARTESIAN_POINT('',(-1.97,2.35,2.4));
#13942=CARTESIAN_POINT('',(-1.97,2.35,2.4));
#13943=CARTESIAN_POINT('',(-1.97,2.35,1.75));
#13944=CARTESIAN_POINT('',(-1.97,2.35,1.75));
#13945=CARTESIAN_POINT('',(-1.97,1.7,1.75));
#13946=CARTESIAN_POINT('',(-1.97,0.78,0.43));
#13947=CARTESIAN_POINT('',(-1.97,0.78,0.43));
#13948=CARTESIAN_POINT('',(-1.97,0.78,1.55));
#13949=CARTESIAN_POINT('',(-1.97,0.78,1.55));
#13950=CARTESIAN_POINT('',(-1.97,-0.78,1.55));
#13951=CARTESIAN_POINT('',(-1.97,-0.78,1.55));
#13952=CARTESIAN_POINT('',(-1.97,-0.78,0.43));
#13953=CARTESIAN_POINT('',(-1.97,-0.78,0.43));
#13954=CARTESIAN_POINT('',(-1.97,-1.7,0.43));
#13955=CARTESIAN_POINT('Origin',(0.,-2.35,1.75));
#13956=CARTESIAN_POINT('',(1.97,-2.35,1.75));
#13957=CARTESIAN_POINT('',(1.97,-2.35,1.75));
#13958=CARTESIAN_POINT('',(0.,-2.35,1.75));
#13959=CARTESIAN_POINT('Origin',(0.,-2.35,2.4));
#13960=CARTESIAN_POINT('',(1.97,-2.35,2.4));
#13961=CARTESIAN_POINT('',(1.97,-2.35,2.4));
#13962=CARTESIAN_POINT('',(0.,-2.35,2.4));
#13963=CARTESIAN_POINT('Origin',(0.,2.35,2.4));
#13964=CARTESIAN_POINT('',(1.97,2.35,2.4));
#13965=CARTESIAN_POINT('',(1.97,2.35,2.4));
#13966=CARTESIAN_POINT('',(0.,2.35,2.4));
#13967=CARTESIAN_POINT('Origin',(0.,2.35,1.75));
#13968=CARTESIAN_POINT('',(1.97,2.35,1.75));
#13969=CARTESIAN_POINT('',(1.97,2.35,1.75));
#13970=CARTESIAN_POINT('',(0.,2.35,1.75));
#13971=CARTESIAN_POINT('Origin',(0.,1.7,1.75));
#13972=CARTESIAN_POINT('',(1.97,1.7,1.75));
#13973=CARTESIAN_POINT('Origin',(0.,0.78,0.43));
#13974=CARTESIAN_POINT('',(1.97,0.78,0.43));
#13975=CARTESIAN_POINT('',(1.97,0.78,0.43));
#13976=CARTESIAN_POINT('',(0.,0.78,0.43));
#13977=CARTESIAN_POINT('Origin',(0.,0.78,1.55));
#13978=CARTESIAN_POINT('',(1.97,0.78,1.55));
#13979=CARTESIAN_POINT('',(1.97,0.78,1.55));
#13980=CARTESIAN_POINT('',(0.,0.78,1.55));
#13981=CARTESIAN_POINT('Origin',(0.,-0.78,1.55));
#13982=CARTESIAN_POINT('',(1.97,-0.78,1.55));
#13983=CARTESIAN_POINT('',(1.97,-0.78,1.55));
#13984=CARTESIAN_POINT('',(0.,-0.78,1.55));
#13985=CARTESIAN_POINT('Origin',(0.,-0.78,0.43));
#13986=CARTESIAN_POINT('',(1.97,-0.78,0.43));
#13987=CARTESIAN_POINT('',(1.97,-0.78,0.43));
#13988=CARTESIAN_POINT('',(0.,-0.78,0.43));
#13989=CARTESIAN_POINT('Origin',(0.,-1.7,0.43));
#13990=CARTESIAN_POINT('',(1.97,-1.7,0.43));
#13991=CARTESIAN_POINT('Origin',(1.97,0.,1.415));
#14437=UNCERTAINTY_MEASURE_WITH_UNIT(LENGTH_MEASURE(0.001),#14479,
'DISTANCE_ACCURACY_VALUE',
'Maximum model space distance between geometric entities at asserted c
onnectivities');
#14446=UNCERTAINTY_MEASURE_WITH_UNIT(LENGTH_MEASURE(0.001),#14479,
'DISTANCE_ACCURACY_VALUE',
'Maximum model space distance between geometric entities at asserted c
onnectivities');
#14469=(
GEOMETRIC_REPRESENTATION_CONTEXT(3)
GLOBAL_UNCERTAINTY_ASSIGNED_CONTEXT((#14437))
GLOBAL_UNIT_ASSIGNED_CONTEXT((#14479,#14481,#14482))
REPRESENTATION_CONTEXT('','3D')
);
#14478=(
GEOMETRIC_REPRESENTATION_CONTEXT(3)
GLOBAL_UNCERTAINTY_ASSIGNED_CONTEXT((#14446))
GLOBAL_UNIT_ASSIGNED_CONTEXT((#14479,#14481,#14482))
REPRESENTATION_CONTEXT('','3D')
);
#14479=(
LENGTH_UNIT()
NAMED_UNIT(*)
SI_UNIT(.CENTI.,.METRE.)
);
#14481=(
NAMED_UNIT(*)
PLANE_ANGLE_UNIT()
SI_UNIT($,.RADIAN.)
);
#14482=(
NAMED_UNIT(*)
SI_UNIT($,.STERADIAN.)
SOLID_ANGLE_UNIT()
);
#14505=SHAPE_DEFINITION_REPRESENTATION(#14536,#14625);
#14536=PRODUCT_DEFINITION_SHAPE('',$,#14657);
#14625=SHAPE_REPRESENTATION('',(#9393),#14469);
#14634=PRODUCT_DEFINITION_CONTEXT('part definition',#14729,'design');
#14657=PRODUCT_DEFINITION('Block','Block',#14688,#14634);
#14688=PRODUCT_DEFINITION_FORMATION('',$,#14753);
#14729=APPLICATION_CONTEXT(
'Core Data for Automotive Mechanical Design Process');
#14730=PRODUCT_CONTEXT('part definition',#14729,'mechanical');
#14753=PRODUCT('Block','Block','Block',(#14730));
#14804=COLOUR_RGB('Dark Blue',0.08,0.2,0.34);
#14805=FILL_AREA_STYLE_COLOUR('',#14804);
#14806=FILL_AREA_STYLE('',(#14805));
#14807=SURFACE_STYLE_FILL_AREA(#14806);
#14808=SURFACE_SIDE_STYLE('',(#14807));
#14809=SURFACE_STYLE_USAGE(.BOTH.,#14808);
#14810=PRESENTATION_STYLE_ASSIGNMENT((#14809));
ENDSEC;
END-ISO-10303-21;
